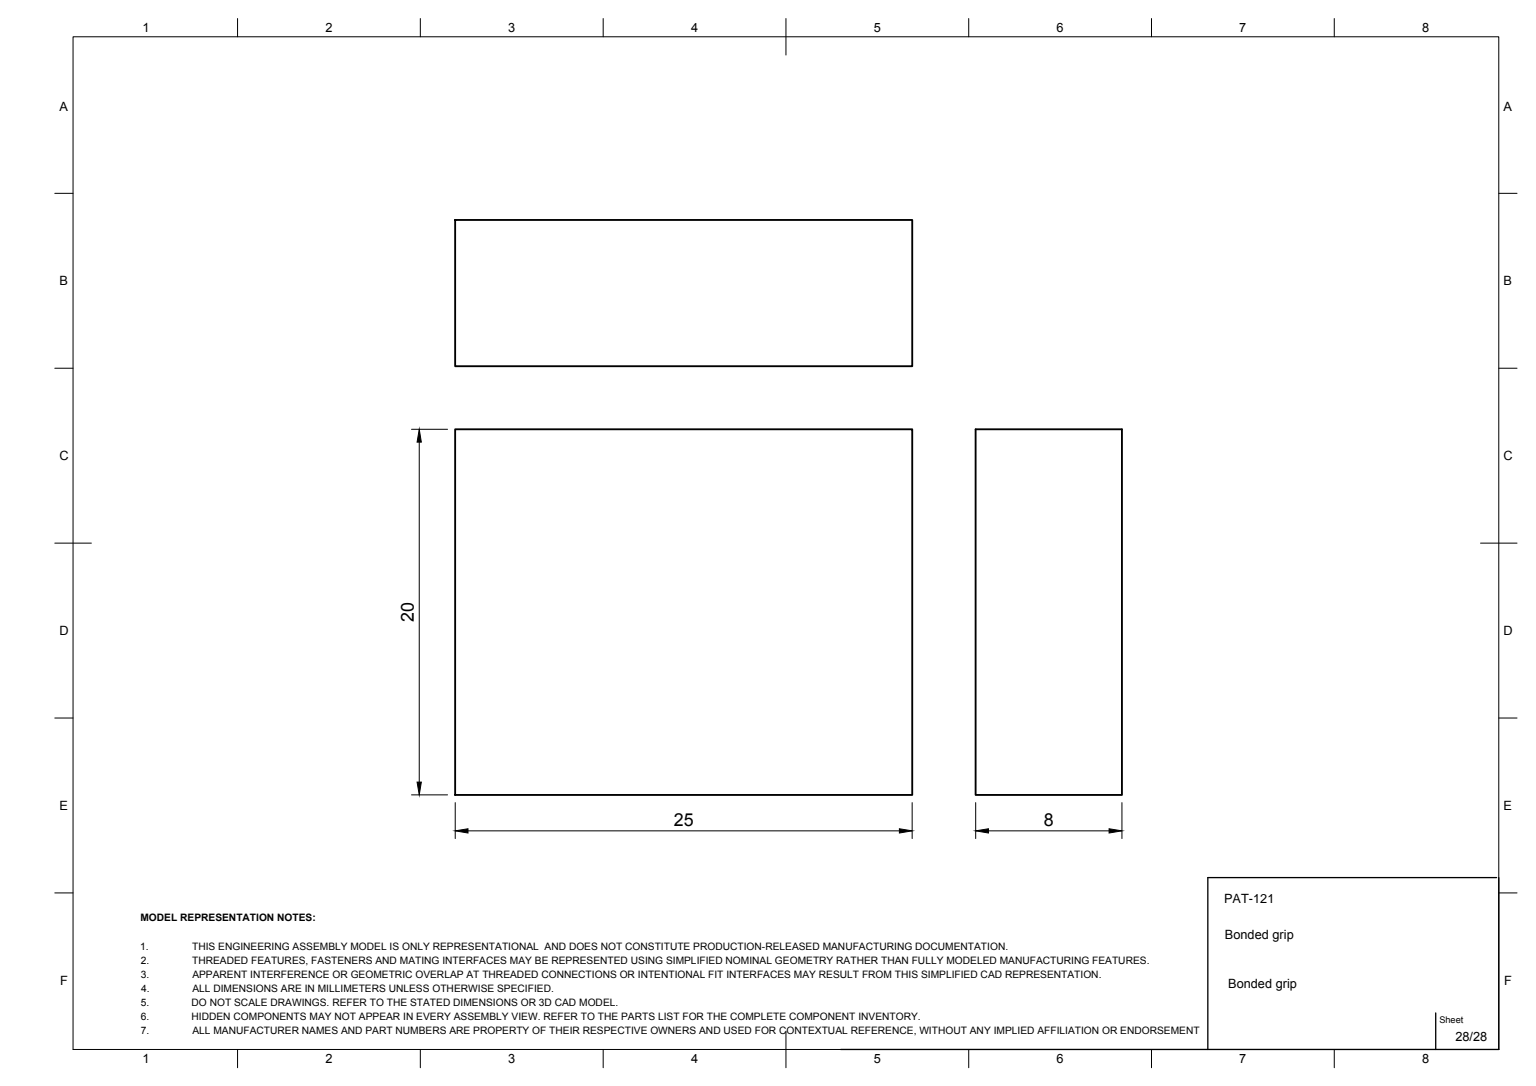
ISO-10303-21;
HEADER;
/* Generated by software containing ST-Developer
 * from STEP Tools, Inc. (www.steptools.com) 
 */

FILE_DESCRIPTION(
/* description */ ('Wall-mounted air drop station'),
/* implementation_level */ '2;1');

FILE_NAME(
/* name */ 'Bonded grip.step',
/* time_stamp */ '2026-10-28T22:16:19-07:00',
/* author */ (''),
/* organization */ (''),
/* preprocessor_version */ 'ST-DEVELOPER v20.2',
/* originating_system */ 'Autodesk Translation Framework v15.17.0.0',
/* authorisation */ '');

FILE_SCHEMA (('AUTOMOTIVE_DESIGN { 1 0 10303 214 3 1 1 }'));
ENDSEC;

DATA;
#10=MECHANICAL_DESIGN_GEOMETRIC_PRESENTATION_REPRESENTATION('',(#371),#10517);
#313=SHAPE_REPRESENTATION_RELATIONSHIP('SRR','None',#10671,#342);
#342=ADVANCED_BREP_SHAPE_REPRESENTATION('',(#398),#10515);
#371=STYLED_ITEM('',(#10881),#398);
#398=MANIFOLD_SOLID_BREP('Body1',#5912);
#738=PLANE('',#6886);
#739=PLANE('',#6887);
#740=PLANE('',#6888);
#741=PLANE('',#6889);
#742=PLANE('',#6890);
#743=PLANE('',#6891);
#1088=FACE_OUTER_BOUND('',#1569,.T.);
#1089=FACE_OUTER_BOUND('',#1570,.T.);
#1090=FACE_OUTER_BOUND('',#1571,.T.);
#1091=FACE_OUTER_BOUND('',#1572,.T.);
#1092=FACE_OUTER_BOUND('',#1573,.T.);
#1093=FACE_OUTER_BOUND('',#1574,.T.);
#1569=EDGE_LOOP('',(#5347,#5348,#5349,#5350));
#1570=EDGE_LOOP('',(#5351,#5352,#5353,#5354));
#1571=EDGE_LOOP('',(#5355,#5356,#5357,#5358));
#1572=EDGE_LOOP('',(#5359,#5360,#5361,#5362));
#1573=EDGE_LOOP('',(#5363,#5364,#5365,#5366));
#1574=EDGE_LOOP('',(#5367,#5368,#5369,#5370));
#2021=LINE('',#10355,#2485);
#2022=LINE('',#10357,#2486);
#2023=LINE('',#10359,#2487);
#2024=LINE('',#10360,#2488);
#2025=LINE('',#10363,#2489);
#2026=LINE('',#10365,#2490);
#2027=LINE('',#10366,#2491);
#2028=LINE('',#10369,#2492);
#2029=LINE('',#10371,#2493);
#2030=LINE('',#10372,#2494);
#2031=LINE('',#10374,#2495);
#2032=LINE('',#10375,#2496);
#2485=VECTOR('',#8657,1.);
#2486=VECTOR('',#8658,1.);
#2487=VECTOR('',#8659,1.);
#2488=VECTOR('',#8660,1.);
#2489=VECTOR('',#8663,1.);
#2490=VECTOR('',#8664,1.);
#2491=VECTOR('',#8665,1.);
#2492=VECTOR('',#8668,1.);
#2493=VECTOR('',#8669,1.);
#2494=VECTOR('',#8670,1.);
#2495=VECTOR('',#8673,1.);
#2496=VECTOR('',#8674,1.);
#3217=VERTEX_POINT('',#10353);
#3218=VERTEX_POINT('',#10354);
#3219=VERTEX_POINT('',#10356);
#3220=VERTEX_POINT('',#10358);
#3221=VERTEX_POINT('',#10362);
#3222=VERTEX_POINT('',#10364);
#3223=VERTEX_POINT('',#10368);
#3224=VERTEX_POINT('',#10370);
#3931=EDGE_CURVE('',#3217,#3218,#2021,.T.);
#3932=EDGE_CURVE('',#3218,#3219,#2022,.T.);
#3933=EDGE_CURVE('',#3220,#3219,#2023,.T.);
#3934=EDGE_CURVE('',#3217,#3220,#2024,.T.);
#3935=EDGE_CURVE('',#3221,#3217,#2025,.T.);
#3936=EDGE_CURVE('',#3222,#3220,#2026,.T.);
#3937=EDGE_CURVE('',#3221,#3222,#2027,.T.);
#3938=EDGE_CURVE('',#3223,#3221,#2028,.T.);
#3939=EDGE_CURVE('',#3224,#3222,#2029,.T.);
#3940=EDGE_CURVE('',#3223,#3224,#2030,.T.);
#3941=EDGE_CURVE('',#3218,#3223,#2031,.T.);
#3942=EDGE_CURVE('',#3219,#3224,#2032,.T.);
#5347=ORIENTED_EDGE('',*,*,#3931,.T.);
#5348=ORIENTED_EDGE('',*,*,#3932,.T.);
#5349=ORIENTED_EDGE('',*,*,#3933,.F.);
#5350=ORIENTED_EDGE('',*,*,#3934,.F.);
#5351=ORIENTED_EDGE('',*,*,#3935,.T.);
#5352=ORIENTED_EDGE('',*,*,#3934,.T.);
#5353=ORIENTED_EDGE('',*,*,#3936,.F.);
#5354=ORIENTED_EDGE('',*,*,#3937,.F.);
#5355=ORIENTED_EDGE('',*,*,#3938,.T.);
#5356=ORIENTED_EDGE('',*,*,#3937,.T.);
#5357=ORIENTED_EDGE('',*,*,#3939,.F.);
#5358=ORIENTED_EDGE('',*,*,#3940,.F.);
#5359=ORIENTED_EDGE('',*,*,#3941,.T.);
#5360=ORIENTED_EDGE('',*,*,#3940,.T.);
#5361=ORIENTED_EDGE('',*,*,#3942,.F.);
#5362=ORIENTED_EDGE('',*,*,#3932,.F.);
#5363=ORIENTED_EDGE('',*,*,#3942,.T.);
#5364=ORIENTED_EDGE('',*,*,#3939,.T.);
#5365=ORIENTED_EDGE('',*,*,#3936,.T.);
#5366=ORIENTED_EDGE('',*,*,#3933,.T.);
#5367=ORIENTED_EDGE('',*,*,#3941,.F.);
#5368=ORIENTED_EDGE('',*,*,#3931,.F.);
#5369=ORIENTED_EDGE('',*,*,#3935,.F.);
#5370=ORIENTED_EDGE('',*,*,#3938,.F.);
#5861=ADVANCED_FACE('',(#1088),#738,.T.);
#5862=ADVANCED_FACE('',(#1089),#739,.T.);
#5863=ADVANCED_FACE('',(#1090),#740,.T.);
#5864=ADVANCED_FACE('',(#1091),#741,.T.);
#5865=ADVANCED_FACE('',(#1092),#742,.T.);
#5866=ADVANCED_FACE('',(#1093),#743,.F.);
#5912=CLOSED_SHELL('',(#5861,#5862,#5863,#5864,#5865,#5866));
#6885=AXIS2_PLACEMENT_3D('',#10351,#8653,#8654);
#6886=AXIS2_PLACEMENT_3D('',#10352,#8655,#8656);
#6887=AXIS2_PLACEMENT_3D('',#10361,#8661,#8662);
#6888=AXIS2_PLACEMENT_3D('',#10367,#8666,#8667);
#6889=AXIS2_PLACEMENT_3D('',#10373,#8671,#8672);
#6890=AXIS2_PLACEMENT_3D('',#10376,#8675,#8676);
#6891=AXIS2_PLACEMENT_3D('',#10377,#8677,#8678);
#8653=DIRECTION('axis',(0.,0.,1.));
#8654=DIRECTION('refdir',(1.,0.,0.));
#8655=DIRECTION('center_axis',(0.,1.,0.));
#8656=DIRECTION('ref_axis',(-1.,0.,0.));
#8657=DIRECTION('',(-1.,0.,0.));
#8658=DIRECTION('',(0.,0.,1.));
#8659=DIRECTION('',(-1.,0.,0.));
#8660=DIRECTION('',(0.,0.,1.));
#8661=DIRECTION('center_axis',(1.,0.,0.));
#8662=DIRECTION('ref_axis',(0.,1.,0.));
#8663=DIRECTION('',(0.,1.,0.));
#8664=DIRECTION('',(0.,1.,0.));
#8665=DIRECTION('',(0.,0.,1.));
#8666=DIRECTION('center_axis',(0.,-1.,0.));
#8667=DIRECTION('ref_axis',(1.,0.,0.));
#8668=DIRECTION('',(1.,0.,0.));
#8669=DIRECTION('',(1.,0.,0.));
#8670=DIRECTION('',(0.,0.,1.));
#8671=DIRECTION('center_axis',(-1.,0.,0.));
#8672=DIRECTION('ref_axis',(0.,-1.,0.));
#8673=DIRECTION('',(0.,-1.,0.));
#8674=DIRECTION('',(0.,-1.,0.));
#8675=DIRECTION('center_axis',(0.,0.,1.));
#8676=DIRECTION('ref_axis',(1.,0.,0.));
#8677=DIRECTION('center_axis',(0.,0.,1.));
#8678=DIRECTION('ref_axis',(1.,0.,0.));
#10351=CARTESIAN_POINT('',(0.,0.,0.));
#10352=CARTESIAN_POINT('Origin',(8.5,1.,9.4));
#10353=CARTESIAN_POINT('',(8.5,1.,9.4));
#10354=CARTESIAN_POINT('',(6.,1.,9.4));
#10355=CARTESIAN_POINT('',(8.5,1.,9.4));
#10356=CARTESIAN_POINT('',(6.,1.,10.2));
#10357=CARTESIAN_POINT('',(6.,1.,9.4));
#10358=CARTESIAN_POINT('',(8.5,1.,10.2));
#10359=CARTESIAN_POINT('',(8.5,1.,10.2));
#10360=CARTESIAN_POINT('',(8.5,1.,9.4));
#10361=CARTESIAN_POINT('Origin',(8.5,-1.,9.4));
#10362=CARTESIAN_POINT('',(8.5,-1.,9.4));
#10363=CARTESIAN_POINT('',(8.5,-1.,9.4));
#10364=CARTESIAN_POINT('',(8.5,-1.,10.2));
#10365=CARTESIAN_POINT('',(8.5,-1.,10.2));
#10366=CARTESIAN_POINT('',(8.5,-1.,9.4));
#10367=CARTESIAN_POINT('Origin',(6.,-1.,9.4));
#10368=CARTESIAN_POINT('',(6.,-1.,9.4));
#10369=CARTESIAN_POINT('',(6.,-1.,9.4));
#10370=CARTESIAN_POINT('',(6.,-1.,10.2));
#10371=CARTESIAN_POINT('',(6.,-1.,10.2));
#10372=CARTESIAN_POINT('',(6.,-1.,9.4));
#10373=CARTESIAN_POINT('Origin',(6.,1.,9.4));
#10374=CARTESIAN_POINT('',(6.,1.,9.4));
#10375=CARTESIAN_POINT('',(6.,1.,10.2));
#10376=CARTESIAN_POINT('Origin',(7.25,0.,10.2));
#10377=CARTESIAN_POINT('Origin',(7.25,0.,9.4));
#10482=UNCERTAINTY_MEASURE_WITH_UNIT(LENGTH_MEASURE(0.001),#10518,
'DISTANCE_ACCURACY_VALUE',
'Maximum model space distance between geometric entities at asserted c
onnectivities');
#10484=UNCERTAINTY_MEASURE_WITH_UNIT(LENGTH_MEASURE(0.001),#10518,
'DISTANCE_ACCURACY_VALUE',
'Maximum model space distance between geometric entities at asserted c
onnectivities');
#10515=(
GEOMETRIC_REPRESENTATION_CONTEXT(3)
GLOBAL_UNCERTAINTY_ASSIGNED_CONTEXT((#10482))
GLOBAL_UNIT_ASSIGNED_CONTEXT((#10518,#10520,#10521))
REPRESENTATION_CONTEXT('','3D')
);
#10517=(
GEOMETRIC_REPRESENTATION_CONTEXT(3)
GLOBAL_UNCERTAINTY_ASSIGNED_CONTEXT((#10484))
GLOBAL_UNIT_ASSIGNED_CONTEXT((#10518,#10520,#10521))
REPRESENTATION_CONTEXT('','3D')
);
#10518=(
LENGTH_UNIT()
NAMED_UNIT(*)
SI_UNIT(.CENTI.,.METRE.)
);
#10520=(
NAMED_UNIT(*)
PLANE_ANGLE_UNIT()
SI_UNIT($,.RADIAN.)
);
#10521=(
NAMED_UNIT(*)
SI_UNIT($,.STERADIAN.)
SOLID_ANGLE_UNIT()
);
#10552=SHAPE_DEFINITION_REPRESENTATION(#10631,#10671);
#10631=PRODUCT_DEFINITION_SHAPE('',$,#10704);
#10671=SHAPE_REPRESENTATION('',(#6885),#10515);
#10673=PRODUCT_DEFINITION_CONTEXT('part definition',#10771,'design');
#10704=PRODUCT_DEFINITION('Bonded grip','Bonded grip',#10736,#10673);
#10736=PRODUCT_DEFINITION_FORMATION('',$,#10803);
#10771=APPLICATION_CONTEXT(
'Core Data for Automotive Mechanical Design Process');
#10772=PRODUCT_CONTEXT('part definition',#10771,'mechanical');
#10803=PRODUCT('Bonded grip','Bonded grip','Bonded grip',(#10772));
#10875=COLOUR_RGB('Black',0.12,0.14,0.17);
#10876=FILL_AREA_STYLE_COLOUR('',#10875);
#10877=FILL_AREA_STYLE('',(#10876));
#10878=SURFACE_STYLE_FILL_AREA(#10877);
#10879=SURFACE_SIDE_STYLE('',(#10878));
#10880=SURFACE_STYLE_USAGE(.BOTH.,#10879);
#10881=PRESENTATION_STYLE_ASSIGNMENT((#10880));
ENDSEC;
END-ISO-10303-21;
